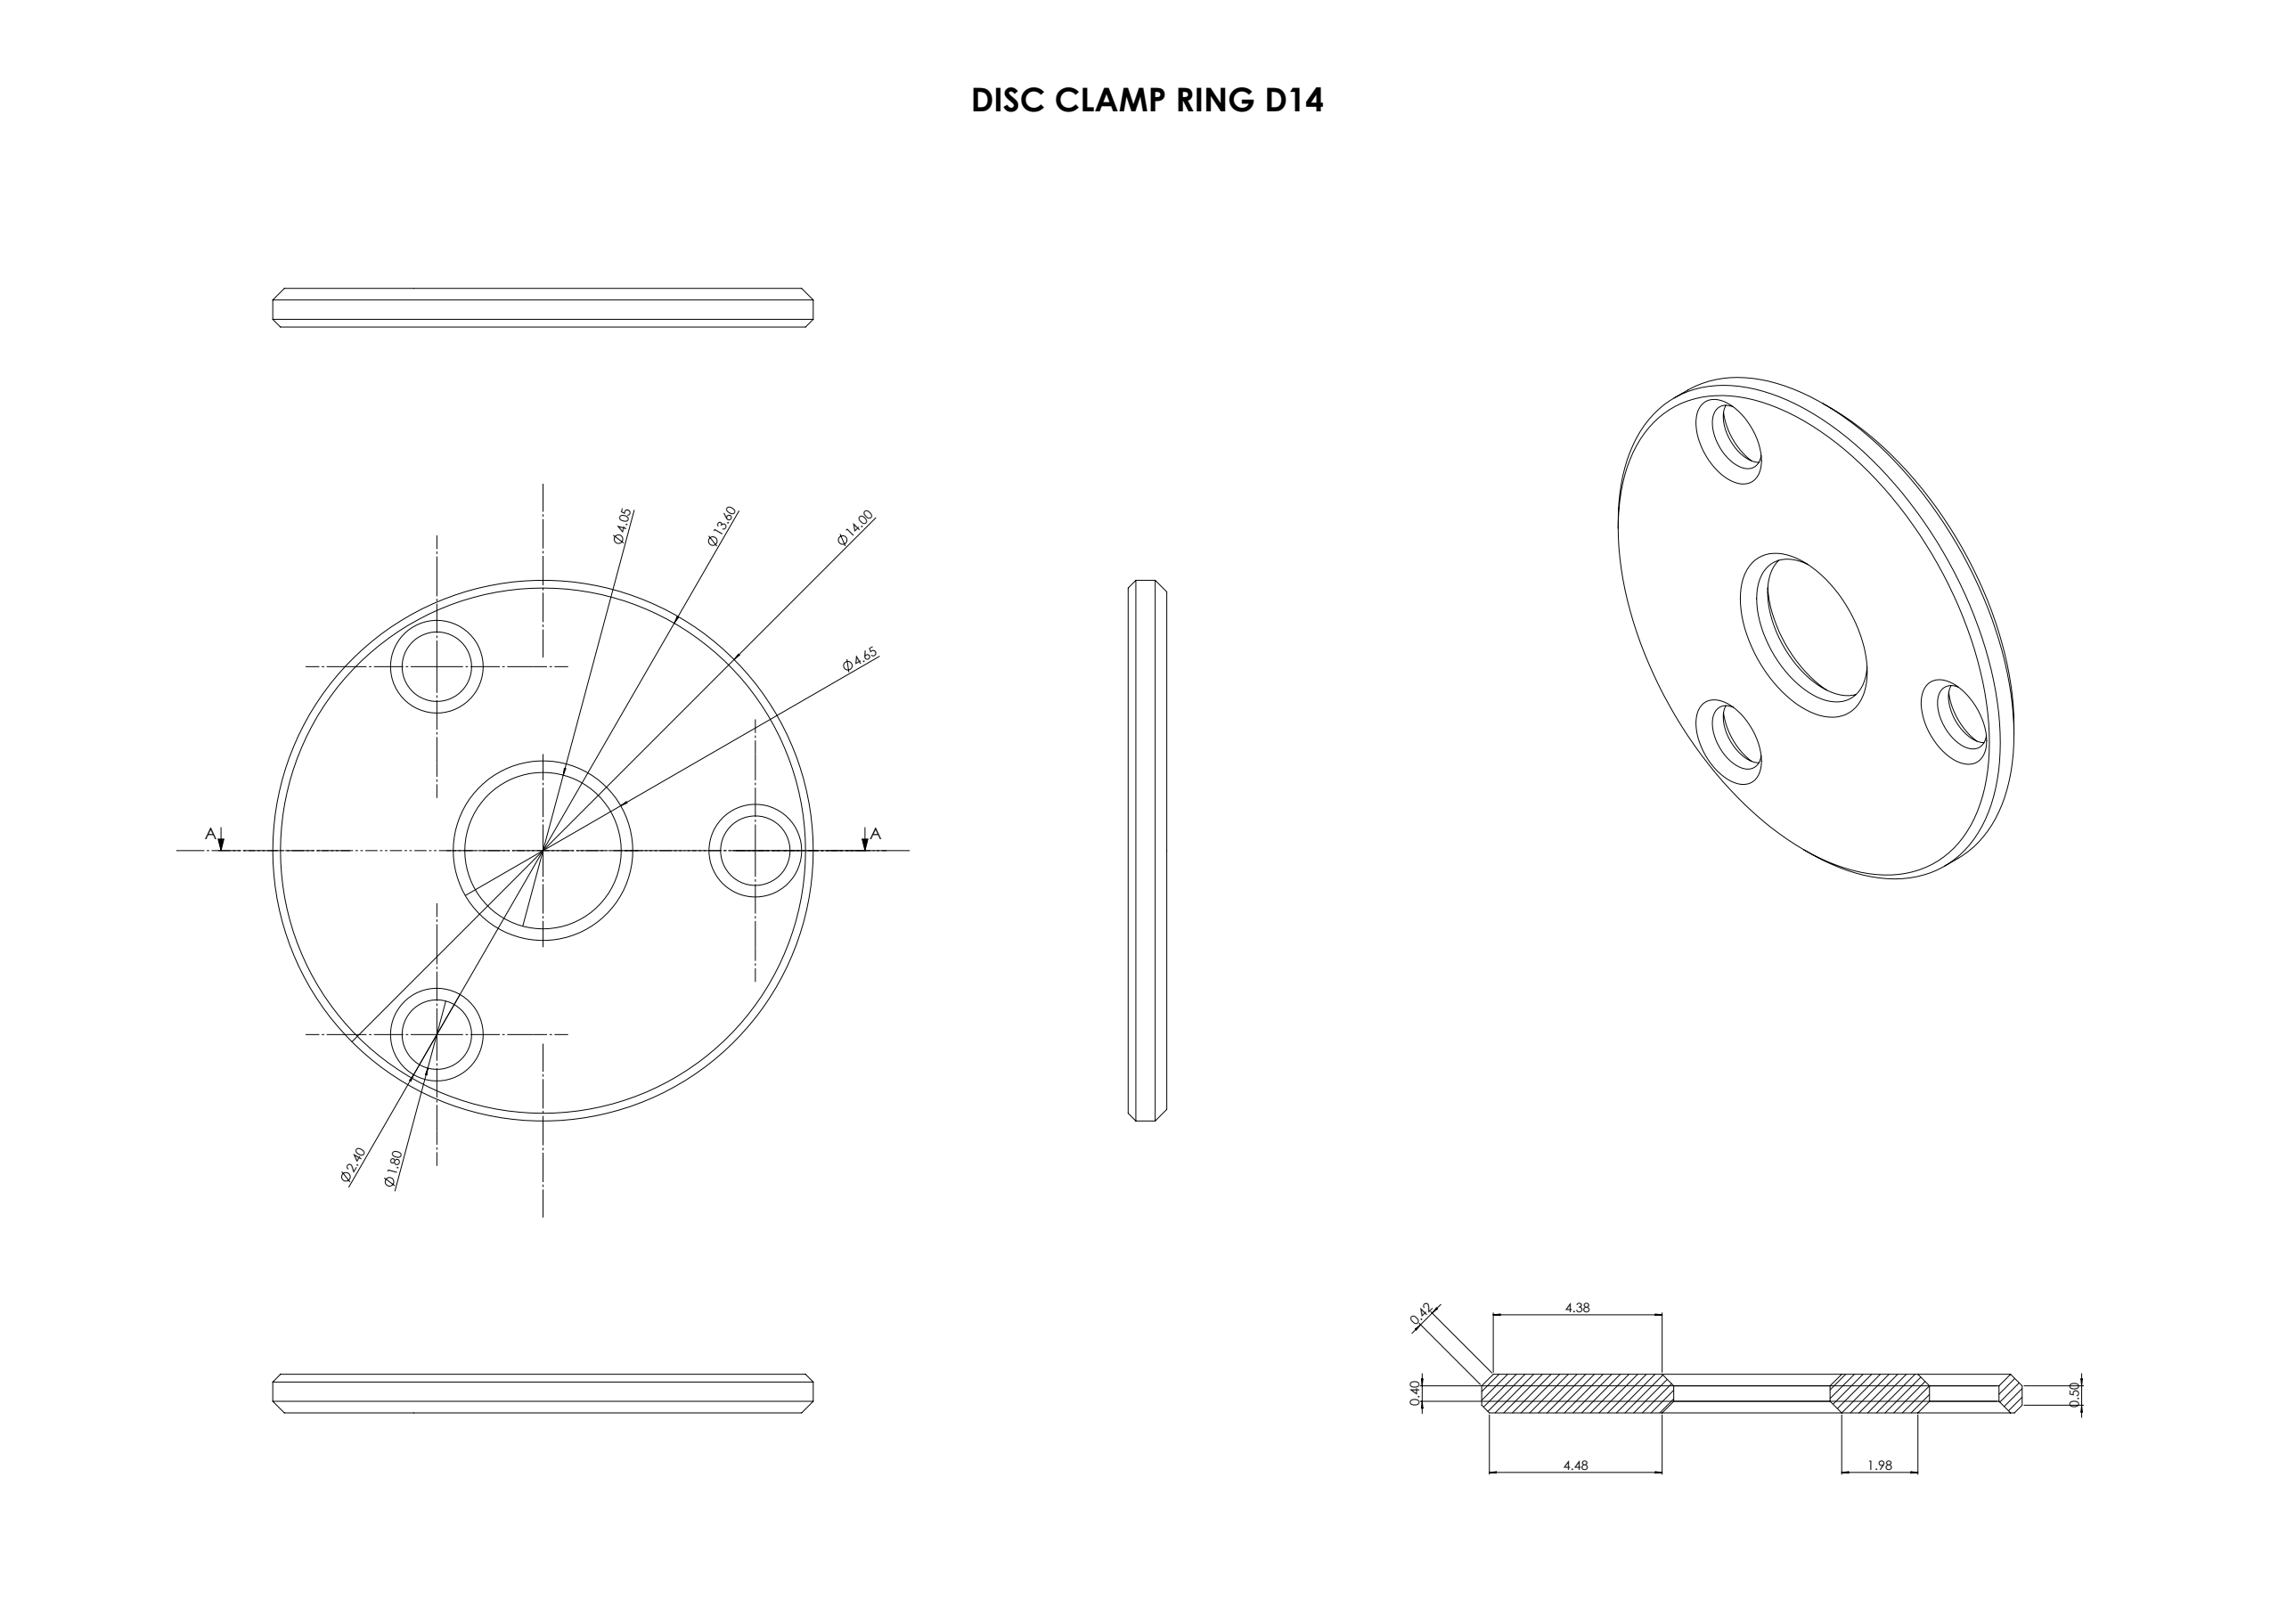
ISO-10303-21;
HEADER;
/* Generated by software containing ST-Developer
 * from STEP Tools, Inc. (www.steptools.com) 
 */

FILE_DESCRIPTION(
/* description */ (''),
/* implementation_level */ '2;1');

FILE_NAME(
/* name */ '09_Disc_Clamp_Ring_D14.step',
/* time_stamp */ '2026-10-19T23:00:43-07:00',
/* author */ (''),
/* organization */ (''),
/* preprocessor_version */ 'ST-DEVELOPER v20.2',
/* originating_system */ 'Autodesk Translation Framework v15.15.0.0',
/* authorisation */ '');

FILE_SCHEMA (('AUTOMOTIVE_DESIGN { 1 0 10303 214 3 1 1 }'));
ENDSEC;

DATA;
#10=MECHANICAL_DESIGN_GEOMETRIC_PRESENTATION_REPRESENTATION('',(#1004),#55002);
#964=SHAPE_REPRESENTATION_RELATIONSHIP('SRR','None',#55112,#984);
#984=ADVANCED_BREP_SHAPE_REPRESENTATION('',(#1024),#54990);
#1004=STYLED_ITEM('',(#55400),#1024);
#1024=MANIFOLD_SOLID_BREP('Disc Clamp Ring',#24537);
#1207=FACE_BOUND('',#4487,.T.);
#1208=FACE_BOUND('',#4490,.T.);
#1209=FACE_BOUND('',#4491,.T.);
#1210=FACE_BOUND('',#4492,.T.);
#1211=FACE_BOUND('',#4493,.T.);
#1439=PLANE('',#25914);
#1440=PLANE('',#25926);
#2156=CYLINDRICAL_SURFACE('',#25911,0.2025);
#2157=CYLINDRICAL_SURFACE('',#25934,0.7);
#2158=CYLINDRICAL_SURFACE('',#25939,0.09);
#2159=CYLINDRICAL_SURFACE('',#25944,0.09);
#2160=CYLINDRICAL_SURFACE('',#25949,0.09);
#2949=FACE_OUTER_BOUND('',#4484,.T.);
#2950=FACE_OUTER_BOUND('',#4485,.T.);
#2951=FACE_OUTER_BOUND('',#4486,.T.);
#2952=FACE_OUTER_BOUND('',#4488,.T.);
#2953=FACE_OUTER_BOUND('',#4489,.T.);
#2954=FACE_OUTER_BOUND('',#4494,.T.);
#2955=FACE_OUTER_BOUND('',#4495,.T.);
#2956=FACE_OUTER_BOUND('',#4496,.T.);
#2957=FACE_OUTER_BOUND('',#4497,.T.);
#2958=FACE_OUTER_BOUND('',#4498,.T.);
#2959=FACE_OUTER_BOUND('',#4499,.T.);
#2960=FACE_OUTER_BOUND('',#4500,.T.);
#2961=FACE_OUTER_BOUND('',#4501,.T.);
#2962=FACE_OUTER_BOUND('',#4502,.T.);
#2963=FACE_OUTER_BOUND('',#4503,.T.);
#2964=FACE_OUTER_BOUND('',#4504,.T.);
#2965=FACE_OUTER_BOUND('',#4505,.T.);
#4484=EDGE_LOOP('',(#18324,#18325,#18326,#18327,#18328));
#4485=EDGE_LOOP('',(#18329,#18330,#18331,#18332,#18333,#18334));
#4486=EDGE_LOOP('',(#18335,#18336,#18337,#18338,#18339,#18340,#18341,#18342,
#18343));
#4487=EDGE_LOOP('',(#18344));
#4488=EDGE_LOOP('',(#18345,#18346,#18347,#18348,#18349));
#4489=EDGE_LOOP('',(#18350));
#4490=EDGE_LOOP('',(#18351));
#4491=EDGE_LOOP('',(#18352));
#4492=EDGE_LOOP('',(#18353));
#4493=EDGE_LOOP('',(#18354));
#4494=EDGE_LOOP('',(#18355,#18356,#18357,#18358,#18359,#18360,#18361));
#4495=EDGE_LOOP('',(#18362,#18363,#18364,#18365,#18366,#18367));
#4496=EDGE_LOOP('',(#18368,#18369,#18370,#18371,#18372));
#4497=EDGE_LOOP('',(#18373,#18374,#18375,#18376));
#4498=EDGE_LOOP('',(#18377,#18378,#18379,#18380));
#4499=EDGE_LOOP('',(#18381,#18382,#18383,#18384,#18385));
#4500=EDGE_LOOP('',(#18386,#18387,#18388,#18389));
#4501=EDGE_LOOP('',(#18390,#18391,#18392,#18393));
#4502=EDGE_LOOP('',(#18394,#18395,#18396,#18397,#18398));
#4503=EDGE_LOOP('',(#18399,#18400,#18401,#18402));
#4504=EDGE_LOOP('',(#18403,#18404,#18405,#18406));
#4505=EDGE_LOOP('',(#18407,#18408,#18409,#18410,#18411));
#5985=LINE('',#36982,#7806);
#5986=LINE('',#36991,#7807);
#5987=LINE('',#37010,#7808);
#5988=LINE('',#37026,#7809);
#5989=LINE('',#37032,#7810);
#5990=LINE('',#37035,#7811);
#5991=LINE('',#37039,#7812);
#5992=LINE('',#37042,#7813);
#5993=LINE('',#37045,#7814);
#5994=LINE('',#37049,#7815);
#5995=LINE('',#37052,#7816);
#5996=LINE('',#37055,#7817);
#5997=LINE('',#37059,#7818);
#5998=LINE('',#37062,#7819);
#5999=LINE('',#37064,#7820);
#7806=VECTOR('',#30079,0.2175);
#7807=VECTOR('',#30090,0.2025);
#7808=VECTOR('',#30113,0.2175);
#7809=VECTOR('',#30132,0.685);
#7810=VECTOR('',#30139,0.7);
#7811=VECTOR('',#30142,0.105);
#7812=VECTOR('',#30147,0.09);
#7813=VECTOR('',#30152,0.105);
#7814=VECTOR('',#30155,0.105);
#7815=VECTOR('',#30160,0.09);
#7816=VECTOR('',#30165,0.105);
#7817=VECTOR('',#30168,0.105);
#7818=VECTOR('',#30173,0.09);
#7819=VECTOR('',#30178,0.105);
#7820=VECTOR('',#30181,0.69);
#9615=CIRCLE('',#25908,0.2325);
#9616=CIRCLE('',#25909,0.2025);
#9617=CIRCLE('',#25910,0.2025);
#9618=CIRCLE('',#25912,0.2025);
#9619=CIRCLE('',#25913,0.2025);
#9620=CIRCLE('',#25915,0.12);
#9621=CIRCLE('',#25916,0.67);
#9622=CIRCLE('',#25917,0.12);
#9623=CIRCLE('',#25918,0.12);
#9624=CIRCLE('',#25919,0.67);
#9625=CIRCLE('',#25920,0.12);
#9626=CIRCLE('',#25921,0.12);
#9627=CIRCLE('',#25922,0.67);
#9628=CIRCLE('',#25923,0.12);
#9629=CIRCLE('',#25925,0.2325);
#9630=CIRCLE('',#25927,0.68);
#9631=CIRCLE('',#25928,0.12);
#9632=CIRCLE('',#25929,0.12);
#9633=CIRCLE('',#25930,0.12);
#9634=CIRCLE('',#25932,0.7);
#9635=CIRCLE('',#25933,0.7);
#9636=CIRCLE('',#25935,0.7);
#9637=CIRCLE('',#25936,0.7);
#9638=CIRCLE('',#25938,0.09);
#9639=CIRCLE('',#25940,0.09);
#9640=CIRCLE('',#25943,0.09);
#9641=CIRCLE('',#25945,0.09);
#9642=CIRCLE('',#25948,0.09);
#9643=CIRCLE('',#25950,0.09);
#10815=VERTEX_POINT('',#36979);
#10816=VERTEX_POINT('',#36981);
#10817=VERTEX_POINT('',#36983);
#10818=VERTEX_POINT('',#36987);
#10819=VERTEX_POINT('',#36988);
#10820=VERTEX_POINT('',#36993);
#10821=VERTEX_POINT('',#36994);
#10822=VERTEX_POINT('',#36996);
#10823=VERTEX_POINT('',#36998);
#10824=VERTEX_POINT('',#37001);
#10825=VERTEX_POINT('',#37003);
#10826=VERTEX_POINT('',#37009);
#10827=VERTEX_POINT('',#37013);
#10828=VERTEX_POINT('',#37015);
#10829=VERTEX_POINT('',#37017);
#10830=VERTEX_POINT('',#37019);
#10831=VERTEX_POINT('',#37022);
#10832=VERTEX_POINT('',#37023);
#10833=VERTEX_POINT('',#37028);
#10834=VERTEX_POINT('',#37029);
#10835=VERTEX_POINT('',#37034);
#10836=VERTEX_POINT('',#37038);
#10837=VERTEX_POINT('',#37044);
#10838=VERTEX_POINT('',#37048);
#10839=VERTEX_POINT('',#37054);
#10840=VERTEX_POINT('',#37058);
#13570=EDGE_CURVE('',#10815,#10815,#9615,.T.);
#13571=EDGE_CURVE('',#10815,#10816,#5985,.T.);
#13572=EDGE_CURVE('',#10816,#10817,#9616,.T.);
#13573=EDGE_CURVE('',#10817,#10816,#9617,.T.);
#13574=EDGE_CURVE('',#10818,#10819,#9618,.T.);
#13575=EDGE_CURVE('',#10819,#10818,#9619,.T.);
#13576=EDGE_CURVE('',#10819,#10817,#5986,.T.);
#13577=EDGE_CURVE('',#10820,#10821,#9620,.T.);
#13578=EDGE_CURVE('',#10822,#10820,#9621,.T.);
#13579=EDGE_CURVE('',#10823,#10822,#9622,.T.);
#13580=EDGE_CURVE('',#10822,#10823,#9623,.T.);
#13581=EDGE_CURVE('',#10824,#10822,#9624,.T.);
#13582=EDGE_CURVE('',#10825,#10824,#9625,.T.);
#13583=EDGE_CURVE('',#10824,#10825,#9626,.T.);
#13584=EDGE_CURVE('',#10820,#10824,#9627,.T.);
#13585=EDGE_CURVE('',#10821,#10820,#9628,.T.);
#13586=EDGE_CURVE('',#10818,#10826,#5987,.T.);
#13587=EDGE_CURVE('',#10826,#10826,#9629,.T.);
#13588=EDGE_CURVE('',#10827,#10827,#9630,.T.);
#13589=EDGE_CURVE('',#10828,#10828,#9631,.T.);
#13590=EDGE_CURVE('',#10829,#10829,#9632,.T.);
#13591=EDGE_CURVE('',#10830,#10830,#9633,.T.);
#13592=EDGE_CURVE('',#10831,#10832,#9634,.T.);
#13593=EDGE_CURVE('',#10832,#10831,#9635,.T.);
#13594=EDGE_CURVE('',#10831,#10822,#5988,.T.);
#13595=EDGE_CURVE('',#10833,#10834,#9636,.T.);
#13596=EDGE_CURVE('',#10834,#10833,#9637,.T.);
#13597=EDGE_CURVE('',#10834,#10832,#5989,.T.);
#13598=EDGE_CURVE('',#10823,#10835,#5990,.T.);
#13599=EDGE_CURVE('',#10835,#10835,#9638,.T.);
#13600=EDGE_CURVE('',#10835,#10836,#5991,.T.);
#13601=EDGE_CURVE('',#10836,#10836,#9639,.T.);
#13602=EDGE_CURVE('',#10828,#10836,#5992,.T.);
#13603=EDGE_CURVE('',#10821,#10837,#5993,.T.);
#13604=EDGE_CURVE('',#10837,#10837,#9640,.T.);
#13605=EDGE_CURVE('',#10837,#10838,#5994,.T.);
#13606=EDGE_CURVE('',#10838,#10838,#9641,.T.);
#13607=EDGE_CURVE('',#10830,#10838,#5995,.T.);
#13608=EDGE_CURVE('',#10825,#10839,#5996,.T.);
#13609=EDGE_CURVE('',#10839,#10839,#9642,.T.);
#13610=EDGE_CURVE('',#10839,#10840,#5997,.T.);
#13611=EDGE_CURVE('',#10840,#10840,#9643,.T.);
#13612=EDGE_CURVE('',#10829,#10840,#5998,.T.);
#13613=EDGE_CURVE('',#10827,#10833,#5999,.T.);
#18324=ORIENTED_EDGE('',*,*,#13570,.T.);
#18325=ORIENTED_EDGE('',*,*,#13571,.T.);
#18326=ORIENTED_EDGE('',*,*,#13572,.T.);
#18327=ORIENTED_EDGE('',*,*,#13573,.T.);
#18328=ORIENTED_EDGE('',*,*,#13571,.F.);
#18329=ORIENTED_EDGE('',*,*,#13574,.F.);
#18330=ORIENTED_EDGE('',*,*,#13575,.F.);
#18331=ORIENTED_EDGE('',*,*,#13576,.T.);
#18332=ORIENTED_EDGE('',*,*,#13572,.F.);
#18333=ORIENTED_EDGE('',*,*,#13573,.F.);
#18334=ORIENTED_EDGE('',*,*,#13576,.F.);
#18335=ORIENTED_EDGE('',*,*,#13577,.F.);
#18336=ORIENTED_EDGE('',*,*,#13578,.F.);
#18337=ORIENTED_EDGE('',*,*,#13579,.F.);
#18338=ORIENTED_EDGE('',*,*,#13580,.F.);
#18339=ORIENTED_EDGE('',*,*,#13581,.F.);
#18340=ORIENTED_EDGE('',*,*,#13582,.F.);
#18341=ORIENTED_EDGE('',*,*,#13583,.F.);
#18342=ORIENTED_EDGE('',*,*,#13584,.F.);
#18343=ORIENTED_EDGE('',*,*,#13585,.F.);
#18344=ORIENTED_EDGE('',*,*,#13570,.F.);
#18345=ORIENTED_EDGE('',*,*,#13574,.T.);
#18346=ORIENTED_EDGE('',*,*,#13575,.T.);
#18347=ORIENTED_EDGE('',*,*,#13586,.T.);
#18348=ORIENTED_EDGE('',*,*,#13587,.T.);
#18349=ORIENTED_EDGE('',*,*,#13586,.F.);
#18350=ORIENTED_EDGE('',*,*,#13588,.F.);
#18351=ORIENTED_EDGE('',*,*,#13589,.F.);
#18352=ORIENTED_EDGE('',*,*,#13590,.F.);
#18353=ORIENTED_EDGE('',*,*,#13591,.F.);
#18354=ORIENTED_EDGE('',*,*,#13587,.F.);
#18355=ORIENTED_EDGE('',*,*,#13592,.T.);
#18356=ORIENTED_EDGE('',*,*,#13593,.T.);
#18357=ORIENTED_EDGE('',*,*,#13594,.T.);
#18358=ORIENTED_EDGE('',*,*,#13578,.T.);
#18359=ORIENTED_EDGE('',*,*,#13584,.T.);
#18360=ORIENTED_EDGE('',*,*,#13581,.T.);
#18361=ORIENTED_EDGE('',*,*,#13594,.F.);
#18362=ORIENTED_EDGE('',*,*,#13595,.F.);
#18363=ORIENTED_EDGE('',*,*,#13596,.F.);
#18364=ORIENTED_EDGE('',*,*,#13597,.T.);
#18365=ORIENTED_EDGE('',*,*,#13592,.F.);
#18366=ORIENTED_EDGE('',*,*,#13593,.F.);
#18367=ORIENTED_EDGE('',*,*,#13597,.F.);
#18368=ORIENTED_EDGE('',*,*,#13580,.T.);
#18369=ORIENTED_EDGE('',*,*,#13598,.T.);
#18370=ORIENTED_EDGE('',*,*,#13599,.T.);
#18371=ORIENTED_EDGE('',*,*,#13598,.F.);
#18372=ORIENTED_EDGE('',*,*,#13579,.T.);
#18373=ORIENTED_EDGE('',*,*,#13599,.F.);
#18374=ORIENTED_EDGE('',*,*,#13600,.T.);
#18375=ORIENTED_EDGE('',*,*,#13601,.F.);
#18376=ORIENTED_EDGE('',*,*,#13600,.F.);
#18377=ORIENTED_EDGE('',*,*,#13589,.T.);
#18378=ORIENTED_EDGE('',*,*,#13602,.T.);
#18379=ORIENTED_EDGE('',*,*,#13601,.T.);
#18380=ORIENTED_EDGE('',*,*,#13602,.F.);
#18381=ORIENTED_EDGE('',*,*,#13577,.T.);
#18382=ORIENTED_EDGE('',*,*,#13603,.T.);
#18383=ORIENTED_EDGE('',*,*,#13604,.T.);
#18384=ORIENTED_EDGE('',*,*,#13603,.F.);
#18385=ORIENTED_EDGE('',*,*,#13585,.T.);
#18386=ORIENTED_EDGE('',*,*,#13604,.F.);
#18387=ORIENTED_EDGE('',*,*,#13605,.T.);
#18388=ORIENTED_EDGE('',*,*,#13606,.F.);
#18389=ORIENTED_EDGE('',*,*,#13605,.F.);
#18390=ORIENTED_EDGE('',*,*,#13591,.T.);
#18391=ORIENTED_EDGE('',*,*,#13607,.T.);
#18392=ORIENTED_EDGE('',*,*,#13606,.T.);
#18393=ORIENTED_EDGE('',*,*,#13607,.F.);
#18394=ORIENTED_EDGE('',*,*,#13583,.T.);
#18395=ORIENTED_EDGE('',*,*,#13608,.T.);
#18396=ORIENTED_EDGE('',*,*,#13609,.T.);
#18397=ORIENTED_EDGE('',*,*,#13608,.F.);
#18398=ORIENTED_EDGE('',*,*,#13582,.T.);
#18399=ORIENTED_EDGE('',*,*,#13609,.F.);
#18400=ORIENTED_EDGE('',*,*,#13610,.T.);
#18401=ORIENTED_EDGE('',*,*,#13611,.F.);
#18402=ORIENTED_EDGE('',*,*,#13610,.F.);
#18403=ORIENTED_EDGE('',*,*,#13590,.T.);
#18404=ORIENTED_EDGE('',*,*,#13612,.T.);
#18405=ORIENTED_EDGE('',*,*,#13611,.T.);
#18406=ORIENTED_EDGE('',*,*,#13612,.F.);
#18407=ORIENTED_EDGE('',*,*,#13588,.T.);
#18408=ORIENTED_EDGE('',*,*,#13613,.T.);
#18409=ORIENTED_EDGE('',*,*,#13595,.T.);
#18410=ORIENTED_EDGE('',*,*,#13596,.T.);
#18411=ORIENTED_EDGE('',*,*,#13613,.F.);
#23121=CONICAL_SURFACE('',#25907,0.2175,0.785398163397459);
#23122=CONICAL_SURFACE('',#25924,0.2175,0.785398163397459);
#23123=CONICAL_SURFACE('',#25931,0.685,0.785398163397459);
#23124=CONICAL_SURFACE('',#25937,0.105,0.785398163397459);
#23125=CONICAL_SURFACE('',#25941,0.105,0.785398163397459);
#23126=CONICAL_SURFACE('',#25942,0.105,0.785398163397459);
#23127=CONICAL_SURFACE('',#25946,0.105,0.785398163397459);
#23128=CONICAL_SURFACE('',#25947,0.105,0.785398163397459);
#23129=CONICAL_SURFACE('',#25951,0.105,0.785398163397459);
#23130=CONICAL_SURFACE('',#25952,0.69,0.785398163397459);
#23702=ADVANCED_FACE('',(#2949),#23121,.F.);
#23703=ADVANCED_FACE('',(#2950),#2156,.F.);
#23704=ADVANCED_FACE('',(#2951,#1207),#1439,.T.);
#23705=ADVANCED_FACE('',(#2952),#23122,.F.);
#23706=ADVANCED_FACE('',(#2953,#1208,#1209,#1210,#1211),#1440,.T.);
#23707=ADVANCED_FACE('',(#2954),#23123,.T.);
#23708=ADVANCED_FACE('',(#2955),#2157,.T.);
#23709=ADVANCED_FACE('',(#2956),#23124,.F.);
#23710=ADVANCED_FACE('',(#2957),#2158,.F.);
#23711=ADVANCED_FACE('',(#2958),#23125,.F.);
#23712=ADVANCED_FACE('',(#2959),#23126,.F.);
#23713=ADVANCED_FACE('',(#2960),#2159,.F.);
#23714=ADVANCED_FACE('',(#2961),#23127,.F.);
#23715=ADVANCED_FACE('',(#2962),#23128,.F.);
#23716=ADVANCED_FACE('',(#2963),#2160,.F.);
#23717=ADVANCED_FACE('',(#2964),#23129,.F.);
#23718=ADVANCED_FACE('',(#2965),#23130,.T.);
#24537=CLOSED_SHELL('',(#23702,#23703,#23704,#23705,#23706,#23707,#23708,
#23709,#23710,#23711,#23712,#23713,#23714,#23715,#23716,#23717,#23718));
#25906=AXIS2_PLACEMENT_3D('',#36977,#30073,#30074);
#25907=AXIS2_PLACEMENT_3D('',#36978,#30075,#30076);
#25908=AXIS2_PLACEMENT_3D('',#36980,#30077,#30078);
#25909=AXIS2_PLACEMENT_3D('',#36984,#30080,#30081);
#25910=AXIS2_PLACEMENT_3D('',#36985,#30082,#30083);
#25911=AXIS2_PLACEMENT_3D('',#36986,#30084,#30085);
#25912=AXIS2_PLACEMENT_3D('',#36989,#30086,#30087);
#25913=AXIS2_PLACEMENT_3D('',#36990,#30088,#30089);
#25914=AXIS2_PLACEMENT_3D('',#36992,#30091,#30092);
#25915=AXIS2_PLACEMENT_3D('',#36995,#30093,#30094);
#25916=AXIS2_PLACEMENT_3D('',#36997,#30095,#30096);
#25917=AXIS2_PLACEMENT_3D('',#36999,#30097,#30098);
#25918=AXIS2_PLACEMENT_3D('',#37000,#30099,#30100);
#25919=AXIS2_PLACEMENT_3D('',#37002,#30101,#30102);
#25920=AXIS2_PLACEMENT_3D('',#37004,#30103,#30104);
#25921=AXIS2_PLACEMENT_3D('',#37005,#30105,#30106);
#25922=AXIS2_PLACEMENT_3D('',#37006,#30107,#30108);
#25923=AXIS2_PLACEMENT_3D('',#37007,#30109,#30110);
#25924=AXIS2_PLACEMENT_3D('',#37008,#30111,#30112);
#25925=AXIS2_PLACEMENT_3D('',#37011,#30114,#30115);
#25926=AXIS2_PLACEMENT_3D('',#37012,#30116,#30117);
#25927=AXIS2_PLACEMENT_3D('',#37014,#30118,#30119);
#25928=AXIS2_PLACEMENT_3D('',#37016,#30120,#30121);
#25929=AXIS2_PLACEMENT_3D('',#37018,#30122,#30123);
#25930=AXIS2_PLACEMENT_3D('',#37020,#30124,#30125);
#25931=AXIS2_PLACEMENT_3D('',#37021,#30126,#30127);
#25932=AXIS2_PLACEMENT_3D('',#37024,#30128,#30129);
#25933=AXIS2_PLACEMENT_3D('',#37025,#30130,#30131);
#25934=AXIS2_PLACEMENT_3D('',#37027,#30133,#30134);
#25935=AXIS2_PLACEMENT_3D('',#37030,#30135,#30136);
#25936=AXIS2_PLACEMENT_3D('',#37031,#30137,#30138);
#25937=AXIS2_PLACEMENT_3D('',#37033,#30140,#30141);
#25938=AXIS2_PLACEMENT_3D('',#37036,#30143,#30144);
#25939=AXIS2_PLACEMENT_3D('',#37037,#30145,#30146);
#25940=AXIS2_PLACEMENT_3D('',#37040,#30148,#30149);
#25941=AXIS2_PLACEMENT_3D('',#37041,#30150,#30151);
#25942=AXIS2_PLACEMENT_3D('',#37043,#30153,#30154);
#25943=AXIS2_PLACEMENT_3D('',#37046,#30156,#30157);
#25944=AXIS2_PLACEMENT_3D('',#37047,#30158,#30159);
#25945=AXIS2_PLACEMENT_3D('',#37050,#30161,#30162);
#25946=AXIS2_PLACEMENT_3D('',#37051,#30163,#30164);
#25947=AXIS2_PLACEMENT_3D('',#37053,#30166,#30167);
#25948=AXIS2_PLACEMENT_3D('',#37056,#30169,#30170);
#25949=AXIS2_PLACEMENT_3D('',#37057,#30171,#30172);
#25950=AXIS2_PLACEMENT_3D('',#37060,#30174,#30175);
#25951=AXIS2_PLACEMENT_3D('',#37061,#30176,#30177);
#25952=AXIS2_PLACEMENT_3D('',#37063,#30179,#30180);
#30073=DIRECTION('axis',(0.,0.,1.));
#30074=DIRECTION('refdir',(1.,0.,0.));
#30075=DIRECTION('center_axis',(0.,0.,-1.));
#30076=DIRECTION('ref_axis',(-1.,0.,0.));
#30077=DIRECTION('center_axis',(0.,0.,-1.));
#30078=DIRECTION('ref_axis',(-1.,0.,0.));
#30079=DIRECTION('',(-0.707106781186555,8.65956056235503E-17,0.70710678118654));
#30080=DIRECTION('center_axis',(0.,0.,1.));
#30081=DIRECTION('ref_axis',(-1.,0.,0.));
#30082=DIRECTION('center_axis',(0.,0.,1.));
#30083=DIRECTION('ref_axis',(-1.,0.,0.));
#30084=DIRECTION('center_axis',(0.,0.,1.));
#30085=DIRECTION('ref_axis',(1.,0.,0.));
#30086=DIRECTION('center_axis',(0.,0.,-1.));
#30087=DIRECTION('ref_axis',(-1.,0.,0.));
#30088=DIRECTION('center_axis',(0.,0.,-1.));
#30089=DIRECTION('ref_axis',(-1.,0.,0.));
#30090=DIRECTION('',(0.,0.,-1.));
#30091=DIRECTION('center_axis',(0.,0.,-1.));
#30092=DIRECTION('ref_axis',(-1.,0.,0.));
#30093=DIRECTION('center_axis',(0.,0.,-1.));
#30094=DIRECTION('ref_axis',(1.,0.,0.));
#30095=DIRECTION('center_axis',(0.,0.,1.));
#30096=DIRECTION('ref_axis',(-1.,0.,0.));
#30097=DIRECTION('center_axis',(0.,0.,-1.));
#30098=DIRECTION('ref_axis',(1.,0.,0.));
#30099=DIRECTION('center_axis',(0.,0.,-1.));
#30100=DIRECTION('ref_axis',(1.,0.,0.));
#30101=DIRECTION('center_axis',(0.,0.,1.));
#30102=DIRECTION('ref_axis',(-1.,0.,0.));
#30103=DIRECTION('center_axis',(0.,0.,-1.));
#30104=DIRECTION('ref_axis',(1.,0.,0.));
#30105=DIRECTION('center_axis',(0.,0.,-1.));
#30106=DIRECTION('ref_axis',(1.,0.,0.));
#30107=DIRECTION('center_axis',(0.,0.,1.));
#30108=DIRECTION('ref_axis',(-1.,0.,0.));
#30109=DIRECTION('center_axis',(0.,0.,-1.));
#30110=DIRECTION('ref_axis',(1.,0.,0.));
#30111=DIRECTION('center_axis',(0.,0.,1.));
#30112=DIRECTION('ref_axis',(-1.,0.,0.));
#30113=DIRECTION('',(0.707106781186555,-8.65956056235503E-17,0.70710678118654));
#30114=DIRECTION('center_axis',(0.,0.,1.));
#30115=DIRECTION('ref_axis',(-1.,0.,0.));
#30116=DIRECTION('center_axis',(0.,0.,1.));
#30117=DIRECTION('ref_axis',(1.,0.,0.));
#30118=DIRECTION('center_axis',(0.,0.,-1.));
#30119=DIRECTION('ref_axis',(-1.,0.,0.));
#30120=DIRECTION('center_axis',(0.,0.,1.));
#30121=DIRECTION('ref_axis',(1.,0.,0.));
#30122=DIRECTION('center_axis',(0.,0.,1.));
#30123=DIRECTION('ref_axis',(1.,0.,0.));
#30124=DIRECTION('center_axis',(0.,0.,1.));
#30125=DIRECTION('ref_axis',(1.,0.,0.));
#30126=DIRECTION('center_axis',(0.,0.,1.));
#30127=DIRECTION('ref_axis',(-1.,0.,0.));
#30128=DIRECTION('center_axis',(0.,0.,-1.));
#30129=DIRECTION('ref_axis',(-1.,0.,0.));
#30130=DIRECTION('center_axis',(0.,0.,-1.));
#30131=DIRECTION('ref_axis',(-1.,0.,0.));
#30132=DIRECTION('',(-0.707106781186555,-8.65956056235503E-17,-0.70710678118654));
#30133=DIRECTION('center_axis',(0.,0.,1.));
#30134=DIRECTION('ref_axis',(1.,0.,0.));
#30135=DIRECTION('center_axis',(0.,0.,1.));
#30136=DIRECTION('ref_axis',(-1.,0.,0.));
#30137=DIRECTION('center_axis',(0.,0.,1.));
#30138=DIRECTION('ref_axis',(-1.,0.,0.));
#30139=DIRECTION('',(0.,0.,-1.));
#30140=DIRECTION('center_axis',(0.,0.,-1.));
#30141=DIRECTION('ref_axis',(1.,0.,0.));
#30142=DIRECTION('',(0.707106781186555,-8.65956056235503E-17,0.70710678118654));
#30143=DIRECTION('center_axis',(0.,0.,1.));
#30144=DIRECTION('ref_axis',(1.,0.,0.));
#30145=DIRECTION('center_axis',(0.,0.,1.));
#30146=DIRECTION('ref_axis',(1.,0.,0.));
#30147=DIRECTION('',(0.,0.,1.));
#30148=DIRECTION('center_axis',(0.,0.,-1.));
#30149=DIRECTION('ref_axis',(1.,0.,0.));
#30150=DIRECTION('center_axis',(0.,0.,1.));
#30151=DIRECTION('ref_axis',(1.,0.,0.));
#30152=DIRECTION('',(0.707106781186555,8.65956056235503E-17,-0.70710678118654));
#30153=DIRECTION('center_axis',(0.,0.,-1.));
#30154=DIRECTION('ref_axis',(1.,0.,0.));
#30155=DIRECTION('',(0.707106781186555,-8.65956056235503E-17,0.70710678118654));
#30156=DIRECTION('center_axis',(0.,0.,1.));
#30157=DIRECTION('ref_axis',(1.,0.,0.));
#30158=DIRECTION('center_axis',(0.,0.,1.));
#30159=DIRECTION('ref_axis',(1.,0.,0.));
#30160=DIRECTION('',(0.,0.,1.));
#30161=DIRECTION('center_axis',(0.,0.,-1.));
#30162=DIRECTION('ref_axis',(1.,0.,0.));
#30163=DIRECTION('center_axis',(0.,0.,1.));
#30164=DIRECTION('ref_axis',(1.,0.,0.));
#30165=DIRECTION('',(0.707106781186555,8.65956056235503E-17,-0.70710678118654));
#30166=DIRECTION('center_axis',(0.,0.,-1.));
#30167=DIRECTION('ref_axis',(1.,0.,0.));
#30168=DIRECTION('',(0.707106781186555,-8.65956056235503E-17,0.70710678118654));
#30169=DIRECTION('center_axis',(0.,0.,1.));
#30170=DIRECTION('ref_axis',(1.,0.,0.));
#30171=DIRECTION('center_axis',(0.,0.,1.));
#30172=DIRECTION('ref_axis',(1.,0.,0.));
#30173=DIRECTION('',(0.,0.,1.));
#30174=DIRECTION('center_axis',(0.,0.,-1.));
#30175=DIRECTION('ref_axis',(1.,0.,0.));
#30176=DIRECTION('center_axis',(0.,0.,1.));
#30177=DIRECTION('ref_axis',(1.,0.,0.));
#30178=DIRECTION('',(0.707106781186555,8.65956056235503E-17,-0.70710678118654));
#30179=DIRECTION('center_axis',(0.,0.,-1.));
#30180=DIRECTION('ref_axis',(-1.,0.,0.));
#30181=DIRECTION('',(0.707106781186555,8.65956056235503E-17,-0.70710678118654));
#36977=CARTESIAN_POINT('',(0.,0.,0.));
#36978=CARTESIAN_POINT('Origin',(0.,0.,10.975));
#36979=CARTESIAN_POINT('',(0.2325,-2.8473038080176E-17,10.96));
#36980=CARTESIAN_POINT('Origin',(0.,0.,10.96));
#36981=CARTESIAN_POINT('',(0.2025,2.47990976827339E-17,10.99));
#36982=CARTESIAN_POINT('',(0.2175,-2.66360678814549E-17,10.975));
#36983=CARTESIAN_POINT('',(-0.2025,-2.47990976827339E-17,10.99));
#36984=CARTESIAN_POINT('Origin',(0.,0.,10.99));
#36985=CARTESIAN_POINT('Origin',(0.,0.,10.99));
#36986=CARTESIAN_POINT('Origin',(0.,0.,11.01));
#36987=CARTESIAN_POINT('',(0.2025,-2.47990976827339E-17,11.03));
#36988=CARTESIAN_POINT('',(-0.2025,-2.47990976827339E-17,11.03));
#36989=CARTESIAN_POINT('Origin',(0.,0.,11.03));
#36990=CARTESIAN_POINT('Origin',(0.,0.,11.03));
#36991=CARTESIAN_POINT('',(-0.2025,-2.47990976827339E-17,11.01));
#36992=CARTESIAN_POINT('Origin',(0.7,0.,10.96));
#36993=CARTESIAN_POINT('',(-0.335,0.580237020535574,10.96));
#36994=CARTESIAN_POINT('',(-0.394999999999999,0.476313972081441,10.96));
#36995=CARTESIAN_POINT('Origin',(-0.275,0.476313972081441,10.96));
#36996=CARTESIAN_POINT('',(0.67,0.,10.96));
#36997=CARTESIAN_POINT('Origin',(0.,0.,10.96));
#36998=CARTESIAN_POINT('',(0.43,1.46957615897682E-17,10.96));
#36999=CARTESIAN_POINT('Origin',(0.55,0.,10.96));
#37000=CARTESIAN_POINT('Origin',(0.55,0.,10.96));
#37001=CARTESIAN_POINT('',(-0.335,-0.580237020535574,10.96));
#37002=CARTESIAN_POINT('Origin',(0.,0.,10.96));
#37003=CARTESIAN_POINT('',(-0.395,-0.476313972081441,10.96));
#37004=CARTESIAN_POINT('Origin',(-0.275,-0.476313972081441,10.96));
#37005=CARTESIAN_POINT('Origin',(-0.275,-0.476313972081441,10.96));
#37006=CARTESIAN_POINT('Origin',(0.,0.,10.96));
#37007=CARTESIAN_POINT('Origin',(-0.275,0.476313972081441,10.96));
#37008=CARTESIAN_POINT('Origin',(0.,0.,11.045));
#37009=CARTESIAN_POINT('',(0.2325,2.8473038080176E-17,11.06));
#37010=CARTESIAN_POINT('',(0.2175,-2.66360678814549E-17,11.045));
#37011=CARTESIAN_POINT('Origin',(0.,0.,11.06));
#37012=CARTESIAN_POINT('Origin',(0.2025,0.,11.06));
#37013=CARTESIAN_POINT('',(0.68,-8.327598234202E-17,11.06));
#37014=CARTESIAN_POINT('Origin',(0.,0.,11.06));
#37015=CARTESIAN_POINT('',(0.43,-1.46957615897682E-17,11.06));
#37016=CARTESIAN_POINT('Origin',(0.55,0.,11.06));
#37017=CARTESIAN_POINT('',(-0.395,-0.476313972081441,11.06));
#37018=CARTESIAN_POINT('Origin',(-0.275,-0.476313972081441,11.06));
#37019=CARTESIAN_POINT('',(-0.395,0.476313972081441,11.06));
#37020=CARTESIAN_POINT('Origin',(-0.275,0.476313972081441,11.06));
#37021=CARTESIAN_POINT('Origin',(0.,0.,10.975));
#37022=CARTESIAN_POINT('',(0.7,-8.57252759403147E-17,10.99));
#37023=CARTESIAN_POINT('',(-0.7,-8.57252759403147E-17,10.99));
#37024=CARTESIAN_POINT('Origin',(0.,0.,10.99));
#37025=CARTESIAN_POINT('Origin',(0.,0.,10.99));
#37026=CARTESIAN_POINT('',(0.685,8.38883057415937E-17,10.975));
#37027=CARTESIAN_POINT('Origin',(0.,0.,11.01));
#37028=CARTESIAN_POINT('',(0.7,8.57252759403147E-17,11.04));
#37029=CARTESIAN_POINT('',(-0.7,-8.57252759403147E-17,11.04));
#37030=CARTESIAN_POINT('Origin',(0.,0.,11.04));
#37031=CARTESIAN_POINT('Origin',(0.,0.,11.04));
#37032=CARTESIAN_POINT('',(-0.7,-8.57252759403147E-17,11.01));
#37033=CARTESIAN_POINT('Origin',(0.55,0.,10.975));
#37034=CARTESIAN_POINT('',(0.46,-1.10218211923262E-17,10.99));
#37035=CARTESIAN_POINT('',(0.445,1.28587913910472E-17,10.975));
#37036=CARTESIAN_POINT('Origin',(0.55,0.,10.99));
#37037=CARTESIAN_POINT('Origin',(0.55,0.,11.025));
#37038=CARTESIAN_POINT('',(0.46,1.10218211923262E-17,11.03));
#37039=CARTESIAN_POINT('',(0.46,-1.10218211923262E-17,11.025));
#37040=CARTESIAN_POINT('Origin',(0.55,0.,11.03));
#37041=CARTESIAN_POINT('Origin',(0.55,0.,11.045));
#37042=CARTESIAN_POINT('',(0.445,-1.28587913910472E-17,11.045));
#37043=CARTESIAN_POINT('Origin',(-0.275,0.476313972081441,10.975));
#37044=CARTESIAN_POINT('',(-0.365,0.476313972081441,10.99));
#37045=CARTESIAN_POINT('',(-0.38,0.476313972081441,10.975));
#37046=CARTESIAN_POINT('Origin',(-0.275,0.476313972081441,10.99));
#37047=CARTESIAN_POINT('Origin',(-0.275,0.476313972081441,11.025));
#37048=CARTESIAN_POINT('',(-0.365,0.476313972081441,11.03));
#37049=CARTESIAN_POINT('',(-0.365,0.476313972081441,11.025));
#37050=CARTESIAN_POINT('Origin',(-0.275,0.476313972081441,11.03));
#37051=CARTESIAN_POINT('Origin',(-0.275,0.476313972081441,11.045));
#37052=CARTESIAN_POINT('',(-0.38,0.476313972081441,11.045));
#37053=CARTESIAN_POINT('Origin',(-0.275,-0.476313972081441,10.975));
#37054=CARTESIAN_POINT('',(-0.365,-0.476313972081441,10.99));
#37055=CARTESIAN_POINT('',(-0.38,-0.476313972081441,10.975));
#37056=CARTESIAN_POINT('Origin',(-0.275,-0.476313972081441,10.99));
#37057=CARTESIAN_POINT('Origin',(-0.275,-0.476313972081441,11.025));
#37058=CARTESIAN_POINT('',(-0.365,-0.476313972081441,11.03));
#37059=CARTESIAN_POINT('',(-0.365,-0.476313972081441,11.025));
#37060=CARTESIAN_POINT('Origin',(-0.275,-0.476313972081441,11.03));
#37061=CARTESIAN_POINT('Origin',(-0.275,-0.476313972081441,11.045));
#37062=CARTESIAN_POINT('',(-0.38,-0.476313972081441,11.045));
#37063=CARTESIAN_POINT('Origin',(0.,0.,11.05));
#37064=CARTESIAN_POINT('',(0.69,8.45006291411674E-17,11.05));
#54968=UNCERTAINTY_MEASURE_WITH_UNIT(LENGTH_MEASURE(0.001),#55003,
'DISTANCE_ACCURACY_VALUE',
'Maximum model space distance between geometric entities at asserted c
onnectivities');
#54980=UNCERTAINTY_MEASURE_WITH_UNIT(LENGTH_MEASURE(0.001),#55003,
'DISTANCE_ACCURACY_VALUE',
'Maximum model space distance between geometric entities at asserted c
onnectivities');
#54990=(
GEOMETRIC_REPRESENTATION_CONTEXT(3)
GLOBAL_UNCERTAINTY_ASSIGNED_CONTEXT((#54968))
GLOBAL_UNIT_ASSIGNED_CONTEXT((#55003,#55005,#55006))
REPRESENTATION_CONTEXT('','3D')
);
#55002=(
GEOMETRIC_REPRESENTATION_CONTEXT(3)
GLOBAL_UNCERTAINTY_ASSIGNED_CONTEXT((#54980))
GLOBAL_UNIT_ASSIGNED_CONTEXT((#55003,#55005,#55006))
REPRESENTATION_CONTEXT('','3D')
);
#55003=(
LENGTH_UNIT()
NAMED_UNIT(*)
SI_UNIT(.CENTI.,.METRE.)
);
#55005=(
NAMED_UNIT(*)
PLANE_ANGLE_UNIT()
SI_UNIT($,.RADIAN.)
);
#55006=(
NAMED_UNIT(*)
SI_UNIT($,.STERADIAN.)
SOLID_ANGLE_UNIT()
);
#55016=SHAPE_DEFINITION_REPRESENTATION(#55037,#55112);
#55037=PRODUCT_DEFINITION_SHAPE('',$,#55134);
#55112=SHAPE_REPRESENTATION('',(#25906),#54990);
#55124=PRODUCT_DEFINITION_CONTEXT('part definition',#55189,'design');
#55134=PRODUCT_DEFINITION('2026-10-18-23-36-24-161',
'09_Disc_Clamp_Ring_D14',#55155,#55124);
#55155=PRODUCT_DEFINITION_FORMATION('',$,#55200);
#55189=APPLICATION_CONTEXT(
'Core Data for Automotive Mechanical Design Process');
#55190=PRODUCT_CONTEXT('part definition',#55189,'mechanical');
#55200=PRODUCT('2026-10-18-23-36-24-161','09_Disc_Clamp_Ring_D14',$,(#55190));
#55394=COLOUR_RGB('Off White',0.89,0.88,0.83);
#55395=FILL_AREA_STYLE_COLOUR('',#55394);
#55396=FILL_AREA_STYLE('',(#55395));
#55397=SURFACE_STYLE_FILL_AREA(#55396);
#55398=SURFACE_SIDE_STYLE('',(#55397));
#55399=SURFACE_STYLE_USAGE(.BOTH.,#55398);
#55400=PRESENTATION_STYLE_ASSIGNMENT((#55399));
ENDSEC;
END-ISO-10303-21;
